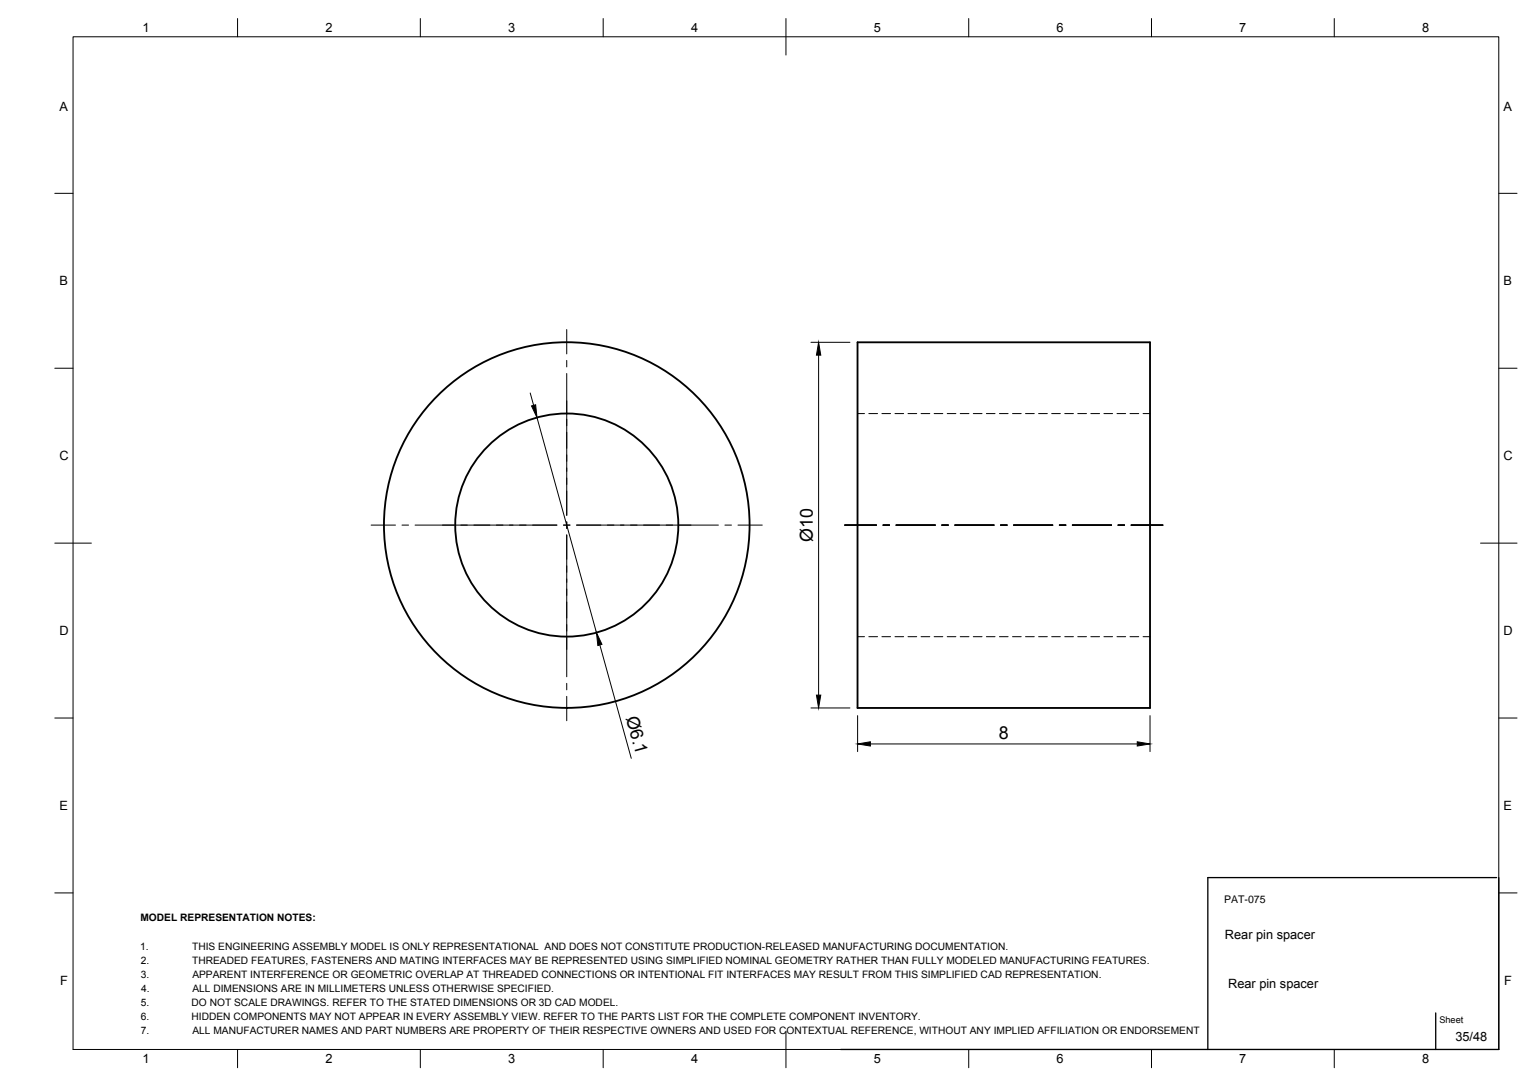
ISO-10303-21;
HEADER;
/* Generated by software containing ST-Developer
 * from STEP Tools, Inc. (www.steptools.com) 
 */

FILE_DESCRIPTION(
/* description */ ('Over-Centre Plunger Toggle Clamp on Slotted Fixture Frame'),
/* implementation_level */ '2;1');

FILE_NAME(
/* name */ 
'Rear pin spacer.step',
/* time_stamp */ '2026-10-28T03:23:24-07:00',
/* author */ (''),
/* organization */ (''),
/* preprocessor_version */ 'ST-DEVELOPER v20.2',
/* originating_system */ 'Autodesk Translation Framework v15.17.0.0',
/* authorisation */ '');

FILE_SCHEMA (('AUTOMOTIVE_DESIGN { 1 0 10303 214 3 1 1 }'));
ENDSEC;

DATA;
#10=MECHANICAL_DESIGN_GEOMETRIC_PRESENTATION_REPRESENTATION('',(#549),#15212);
#457=SHAPE_REPRESENTATION_RELATIONSHIP('SRR','None',#15434,#499);
#499=ADVANCED_BREP_SHAPE_REPRESENTATION('',(#598),#15196);
#549=STYLED_ITEM('',(#15719),#598);
#598=MANIFOLD_SOLID_BREP('Body1',#8283);
#757=FACE_BOUND('',#2088,.T.);
#758=FACE_BOUND('',#2090,.T.);
#1007=PLANE('',#9471);
#1008=PLANE('',#9472);
#1453=FACE_OUTER_BOUND('',#2085,.T.);
#1454=FACE_OUTER_BOUND('',#2086,.T.);
#1455=FACE_OUTER_BOUND('',#2087,.T.);
#1456=FACE_OUTER_BOUND('',#2089,.T.);
#2085=EDGE_LOOP('',(#7159,#7160,#7161,#7162));
#2086=EDGE_LOOP('',(#7163,#7164,#7165,#7166));
#2087=EDGE_LOOP('',(#7167));
#2088=EDGE_LOOP('',(#7168));
#2089=EDGE_LOOP('',(#7169));
#2090=EDGE_LOOP('',(#7170));
#2709=LINE('',#14507,#3339);
#2710=LINE('',#14513,#3340);
#3339=VECTOR('',#11640,0.305);
#3340=VECTOR('',#11647,0.5);
#3784=CIRCLE('',#9466,0.305);
#3785=CIRCLE('',#9467,0.305);
#3786=CIRCLE('',#9469,0.5);
#3787=CIRCLE('',#9470,0.5);
#4396=VERTEX_POINT('',#14504);
#4397=VERTEX_POINT('',#14506);
#4398=VERTEX_POINT('',#14510);
#4399=VERTEX_POINT('',#14512);
#5340=EDGE_CURVE('',#4396,#4396,#3784,.T.);
#5341=EDGE_CURVE('',#4396,#4397,#2709,.T.);
#5342=EDGE_CURVE('',#4397,#4397,#3785,.T.);
#5343=EDGE_CURVE('',#4398,#4398,#3786,.T.);
#5344=EDGE_CURVE('',#4398,#4399,#2710,.T.);
#5345=EDGE_CURVE('',#4399,#4399,#3787,.T.);
#7159=ORIENTED_EDGE('',*,*,#5340,.F.);
#7160=ORIENTED_EDGE('',*,*,#5341,.T.);
#7161=ORIENTED_EDGE('',*,*,#5342,.T.);
#7162=ORIENTED_EDGE('',*,*,#5341,.F.);
#7163=ORIENTED_EDGE('',*,*,#5343,.F.);
#7164=ORIENTED_EDGE('',*,*,#5344,.T.);
#7165=ORIENTED_EDGE('',*,*,#5345,.T.);
#7166=ORIENTED_EDGE('',*,*,#5344,.F.);
#7167=ORIENTED_EDGE('',*,*,#5343,.T.);
#7168=ORIENTED_EDGE('',*,*,#5340,.T.);
#7169=ORIENTED_EDGE('',*,*,#5345,.F.);
#7170=ORIENTED_EDGE('',*,*,#5342,.F.);
#7729=CYLINDRICAL_SURFACE('',#9465,0.305);
#7730=CYLINDRICAL_SURFACE('',#9468,0.5);
#8125=ADVANCED_FACE('',(#1453),#7729,.F.);
#8126=ADVANCED_FACE('',(#1454),#7730,.T.);
#8127=ADVANCED_FACE('',(#1455,#757),#1007,.T.);
#8128=ADVANCED_FACE('',(#1456,#758),#1008,.F.);
#8283=CLOSED_SHELL('',(#8125,#8126,#8127,#8128));
#9464=AXIS2_PLACEMENT_3D('',#14502,#11634,#11635);
#9465=AXIS2_PLACEMENT_3D('',#14503,#11636,#11637);
#9466=AXIS2_PLACEMENT_3D('',#14505,#11638,#11639);
#9467=AXIS2_PLACEMENT_3D('',#14508,#11641,#11642);
#9468=AXIS2_PLACEMENT_3D('',#14509,#11643,#11644);
#9469=AXIS2_PLACEMENT_3D('',#14511,#11645,#11646);
#9470=AXIS2_PLACEMENT_3D('',#14514,#11648,#11649);
#9471=AXIS2_PLACEMENT_3D('',#14515,#11650,#11651);
#9472=AXIS2_PLACEMENT_3D('',#14516,#11652,#11653);
#11634=DIRECTION('axis',(0.,0.,1.));
#11635=DIRECTION('refdir',(1.,0.,0.));
#11636=DIRECTION('center_axis',(0.,1.,0.));
#11637=DIRECTION('ref_axis',(1.,0.,0.));
#11638=DIRECTION('center_axis',(0.,-1.,0.));
#11639=DIRECTION('ref_axis',(1.,0.,0.));
#11640=DIRECTION('',(0.,-1.,0.));
#11641=DIRECTION('center_axis',(0.,-1.,0.));
#11642=DIRECTION('ref_axis',(1.,0.,0.));
#11643=DIRECTION('center_axis',(0.,1.,0.));
#11644=DIRECTION('ref_axis',(1.,0.,0.));
#11645=DIRECTION('center_axis',(0.,1.,0.));
#11646=DIRECTION('ref_axis',(1.,0.,0.));
#11647=DIRECTION('',(0.,-1.,0.));
#11648=DIRECTION('center_axis',(0.,1.,0.));
#11649=DIRECTION('ref_axis',(1.,0.,0.));
#11650=DIRECTION('center_axis',(0.,1.,0.));
#11651=DIRECTION('ref_axis',(1.,0.,0.));
#11652=DIRECTION('center_axis',(0.,1.,0.));
#11653=DIRECTION('ref_axis',(1.,0.,0.));
#14502=CARTESIAN_POINT('',(0.,0.,0.));
#14503=CARTESIAN_POINT('Origin',(-2.82632109303527,-4.7,8.79263101785268));
#14504=CARTESIAN_POINT('',(-3.13132109303527,-3.9,8.79263101785268));
#14505=CARTESIAN_POINT('Origin',(-2.82632109303527,-3.9,8.79263101785268));
#14506=CARTESIAN_POINT('',(-3.13132109303527,-4.7,8.79263101785268));
#14507=CARTESIAN_POINT('',(-3.13132109303527,-4.7,8.79263101785268));
#14508=CARTESIAN_POINT('Origin',(-2.82632109303527,-4.7,8.79263101785268));
#14509=CARTESIAN_POINT('Origin',(-2.82632109303527,-4.7,8.79263101785268));
#14510=CARTESIAN_POINT('',(-3.32632109303527,-3.9,8.79263101785268));
#14511=CARTESIAN_POINT('Origin',(-2.82632109303527,-3.9,8.79263101785268));
#14512=CARTESIAN_POINT('',(-3.32632109303527,-4.7,8.79263101785268));
#14513=CARTESIAN_POINT('',(-3.32632109303527,-4.7,8.79263101785268));
#14514=CARTESIAN_POINT('Origin',(-2.82632109303527,-4.7,8.79263101785268));
#14515=CARTESIAN_POINT('Origin',(-2.82632109303527,-3.9,8.79263101785268));
#14516=CARTESIAN_POINT('Origin',(-2.82632109303527,-4.7,8.79263101785268));
#15146=UNCERTAINTY_MEASURE_WITH_UNIT(LENGTH_MEASURE(0.001),#15213,
'DISTANCE_ACCURACY_VALUE',
'Maximum model space distance between geometric entities at asserted c
onnectivities');
#15162=UNCERTAINTY_MEASURE_WITH_UNIT(LENGTH_MEASURE(0.001),#15213,
'DISTANCE_ACCURACY_VALUE',
'Maximum model space distance between geometric entities at asserted c
onnectivities');
#15196=(
GEOMETRIC_REPRESENTATION_CONTEXT(3)
GLOBAL_UNCERTAINTY_ASSIGNED_CONTEXT((#15146))
GLOBAL_UNIT_ASSIGNED_CONTEXT((#15213,#15215,#15216))
REPRESENTATION_CONTEXT('','3D')
);
#15212=(
GEOMETRIC_REPRESENTATION_CONTEXT(3)
GLOBAL_UNCERTAINTY_ASSIGNED_CONTEXT((#15162))
GLOBAL_UNIT_ASSIGNED_CONTEXT((#15213,#15215,#15216))
REPRESENTATION_CONTEXT('','3D')
);
#15213=(
LENGTH_UNIT()
NAMED_UNIT(*)
SI_UNIT(.CENTI.,.METRE.)
);
#15215=(
NAMED_UNIT(*)
PLANE_ANGLE_UNIT()
SI_UNIT($,.RADIAN.)
);
#15216=(
NAMED_UNIT(*)
SI_UNIT($,.STERADIAN.)
SOLID_ANGLE_UNIT()
);
#15250=SHAPE_DEFINITION_REPRESENTATION(#15306,#15434);
#15306=PRODUCT_DEFINITION_SHAPE('',$,#15484);
#15434=SHAPE_REPRESENTATION('',(#9464),#15196);
#15450=PRODUCT_DEFINITION_CONTEXT('part definition',#15599,'design');
#15484=PRODUCT_DEFINITION('Rear pin spacer','Rear pin spacer',#15533,#15450);
#15533=PRODUCT_DEFINITION_FORMATION('',$,#15634);
#15599=APPLICATION_CONTEXT(
'Core Data for Automotive Mechanical Design Process');
#15600=PRODUCT_CONTEXT('part definition',#15599,'mechanical');
#15634=PRODUCT('Rear pin spacer','Rear pin spacer','Rear pin spacer',(#15600));
#15713=COLOUR_RGB('Grey',0.48,0.52,0.57);
#15714=FILL_AREA_STYLE_COLOUR('',#15713);
#15715=FILL_AREA_STYLE('',(#15714));
#15716=SURFACE_STYLE_FILL_AREA(#15715);
#15717=SURFACE_SIDE_STYLE('',(#15716));
#15718=SURFACE_STYLE_USAGE(.BOTH.,#15717);
#15719=PRESENTATION_STYLE_ASSIGNMENT((#15718));
ENDSEC;
END-ISO-10303-21;
